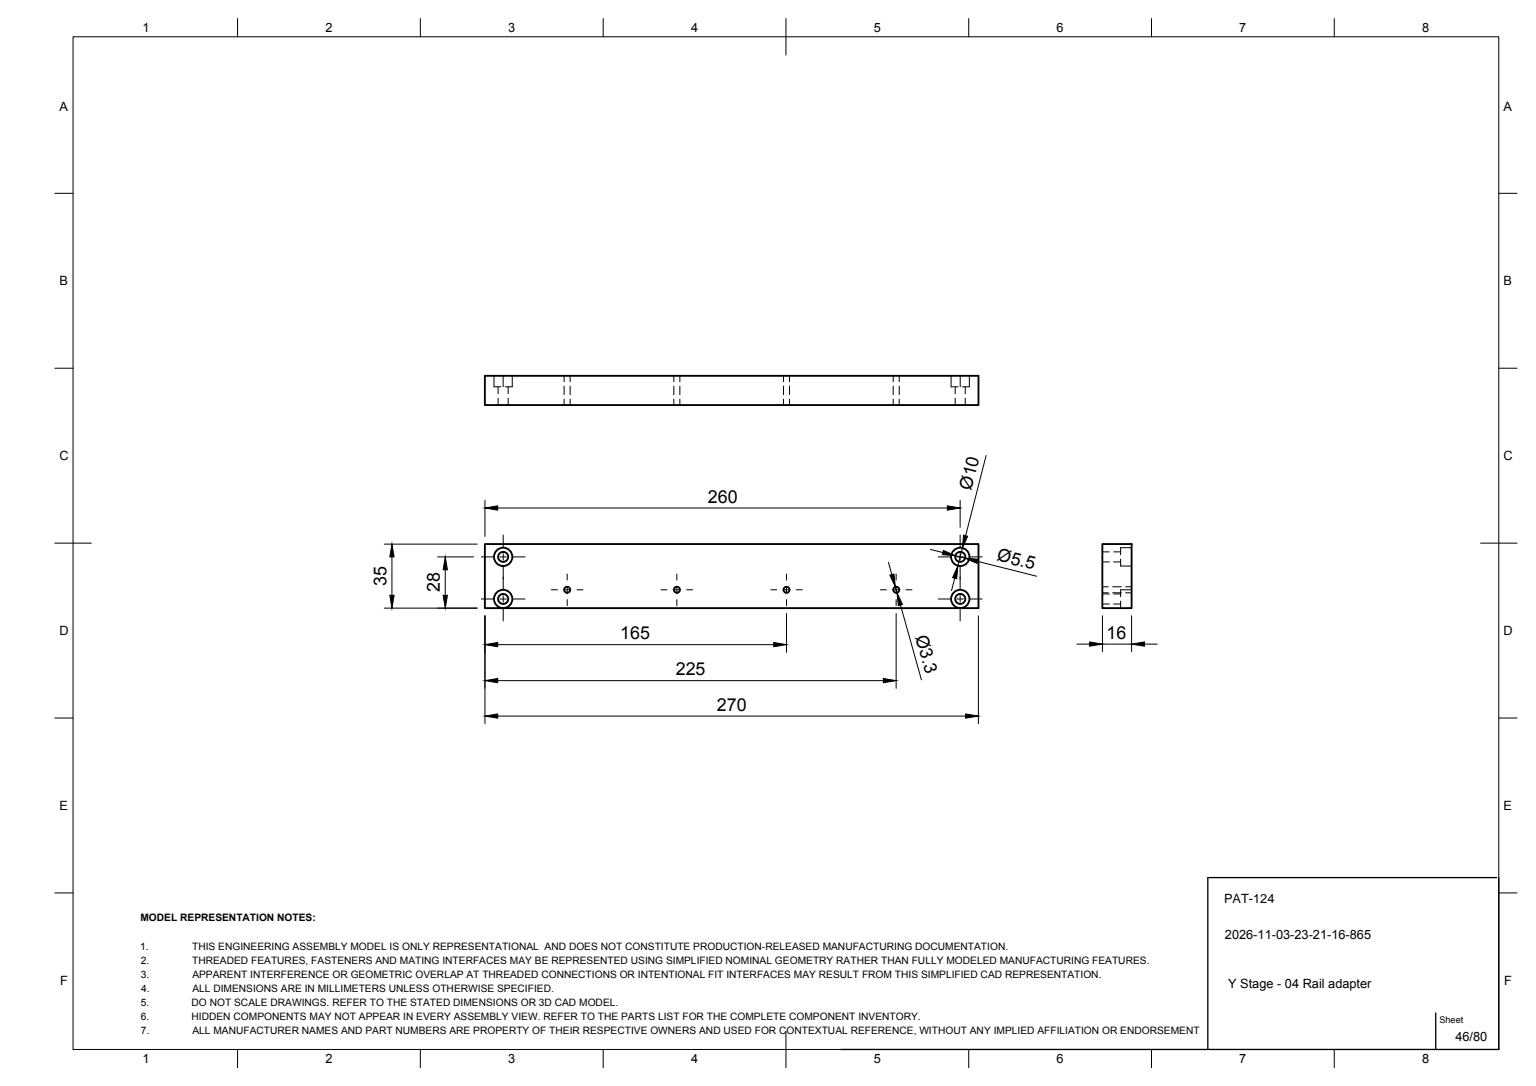
ISO-10303-21;
HEADER;
/* Generated by software containing ST-Developer
 * from STEP Tools, Inc. (www.steptools.com) 
 */

FILE_DESCRIPTION(
/* description */ ('XY cross-slide table'),
/* implementation_level */ '2;1');

FILE_NAME(
/* name */ 'Y Stage - 04 Rail adapter.step',
/* time_stamp */ '2026-10-28T03:22:46-07:00',
/* author */ (''),
/* organization */ (''),
/* preprocessor_version */ 'ST-DEVELOPER v20.2',
/* originating_system */ 'Autodesk Translation Framework v15.17.0.0',
/* authorisation */ '');

FILE_SCHEMA (('AUTOMOTIVE_DESIGN { 1 0 10303 214 3 1 1 }'));
ENDSEC;

DATA;
#10=MECHANICAL_DESIGN_GEOMETRIC_PRESENTATION_REPRESENTATION('',(#1728),#62984);
#1547=SHAPE_REPRESENTATION_RELATIONSHIP('SRR','None',#63402,#1630);
#1630=ADVANCED_BREP_SHAPE_REPRESENTATION('',(#1837),#62939);
#1728=STYLED_ITEM('',(#63905),#1837);
#1837=MANIFOLD_SOLID_BREP('Body1',#23026);
#2125=FACE_BOUND('',#5116,.T.);
#2126=FACE_BOUND('',#5119,.T.);
#2127=FACE_BOUND('',#5122,.T.);
#2128=FACE_BOUND('',#5125,.T.);
#2129=FACE_BOUND('',#5127,.T.);
#2130=FACE_BOUND('',#5128,.T.);
#2131=FACE_BOUND('',#5129,.T.);
#2132=FACE_BOUND('',#5130,.T.);
#2133=FACE_BOUND('',#5131,.T.);
#2134=FACE_BOUND('',#5132,.T.);
#2135=FACE_BOUND('',#5142,.T.);
#2136=FACE_BOUND('',#5143,.T.);
#2137=FACE_BOUND('',#5144,.T.);
#2138=FACE_BOUND('',#5145,.T.);
#2139=FACE_BOUND('',#5146,.T.);
#2140=FACE_BOUND('',#5147,.T.);
#2141=FACE_BOUND('',#5148,.T.);
#2142=FACE_BOUND('',#5149,.T.);
#2595=PLANE('',#25321);
#2596=PLANE('',#25326);
#2597=PLANE('',#25331);
#2598=PLANE('',#25336);
#2599=PLANE('',#25338);
#2600=PLANE('',#25347);
#2601=PLANE('',#25348);
#2602=PLANE('',#25349);
#2603=PLANE('',#25350);
#2604=PLANE('',#25351);
#3556=FACE_OUTER_BOUND('',#5108,.T.);
#3557=FACE_OUTER_BOUND('',#5109,.T.);
#3558=FACE_OUTER_BOUND('',#5110,.T.);
#3559=FACE_OUTER_BOUND('',#5111,.T.);
#3560=FACE_OUTER_BOUND('',#5112,.T.);
#3561=FACE_OUTER_BOUND('',#5113,.T.);
#3562=FACE_OUTER_BOUND('',#5114,.T.);
#3563=FACE_OUTER_BOUND('',#5115,.T.);
#3564=FACE_OUTER_BOUND('',#5117,.T.);
#3565=FACE_OUTER_BOUND('',#5118,.T.);
#3566=FACE_OUTER_BOUND('',#5120,.T.);
#3567=FACE_OUTER_BOUND('',#5121,.T.);
#3568=FACE_OUTER_BOUND('',#5123,.T.);
#3569=FACE_OUTER_BOUND('',#5124,.T.);
#3570=FACE_OUTER_BOUND('',#5126,.T.);
#3571=FACE_OUTER_BOUND('',#5133,.T.);
#3572=FACE_OUTER_BOUND('',#5134,.T.);
#3573=FACE_OUTER_BOUND('',#5135,.T.);
#3574=FACE_OUTER_BOUND('',#5136,.T.);
#3575=FACE_OUTER_BOUND('',#5137,.T.);
#3576=FACE_OUTER_BOUND('',#5138,.T.);
#3577=FACE_OUTER_BOUND('',#5139,.T.);
#3578=FACE_OUTER_BOUND('',#5140,.T.);
#3579=FACE_OUTER_BOUND('',#5141,.T.);
#5108=EDGE_LOOP('',(#18110,#18111,#18112,#18113));
#5109=EDGE_LOOP('',(#18114,#18115,#18116,#18117));
#5110=EDGE_LOOP('',(#18118,#18119,#18120,#18121));
#5111=EDGE_LOOP('',(#18122,#18123,#18124,#18125));
#5112=EDGE_LOOP('',(#18126,#18127,#18128,#18129));
#5113=EDGE_LOOP('',(#18130,#18131,#18132,#18133));
#5114=EDGE_LOOP('',(#18134,#18135,#18136,#18137));
#5115=EDGE_LOOP('',(#18138));
#5116=EDGE_LOOP('',(#18139));
#5117=EDGE_LOOP('',(#18140,#18141,#18142,#18143));
#5118=EDGE_LOOP('',(#18144,#18145));
#5119=EDGE_LOOP('',(#18146));
#5120=EDGE_LOOP('',(#18147,#18148,#18149,#18150));
#5121=EDGE_LOOP('',(#18151));
#5122=EDGE_LOOP('',(#18152));
#5123=EDGE_LOOP('',(#18153,#18154,#18155,#18156));
#5124=EDGE_LOOP('',(#18157,#18158));
#5125=EDGE_LOOP('',(#18159));
#5126=EDGE_LOOP('',(#18160,#18161,#18162,#18163,#18164,#18165,#18166,#18167,
#18168,#18169));
#5127=EDGE_LOOP('',(#18170));
#5128=EDGE_LOOP('',(#18171));
#5129=EDGE_LOOP('',(#18172));
#5130=EDGE_LOOP('',(#18173));
#5131=EDGE_LOOP('',(#18174));
#5132=EDGE_LOOP('',(#18175));
#5133=EDGE_LOOP('',(#18176,#18177,#18178,#18179));
#5134=EDGE_LOOP('',(#18180,#18181,#18182,#18183));
#5135=EDGE_LOOP('',(#18184,#18185,#18186,#18187));
#5136=EDGE_LOOP('',(#18188,#18189,#18190,#18191));
#5137=EDGE_LOOP('',(#18192,#18193,#18194,#18195,#18196,#18197,#18198,#18199,
#18200,#18201));
#5138=EDGE_LOOP('',(#18202,#18203,#18204,#18205));
#5139=EDGE_LOOP('',(#18206,#18207,#18208,#18209));
#5140=EDGE_LOOP('',(#18210,#18211,#18212,#18213));
#5141=EDGE_LOOP('',(#18214,#18215,#18216,#18217));
#5142=EDGE_LOOP('',(#18218));
#5143=EDGE_LOOP('',(#18219));
#5144=EDGE_LOOP('',(#18220));
#5145=EDGE_LOOP('',(#18221));
#5146=EDGE_LOOP('',(#18222));
#5147=EDGE_LOOP('',(#18223));
#5148=EDGE_LOOP('',(#18224));
#5149=EDGE_LOOP('',(#18225));
#6682=LINE('',#47980,#8169);
#6683=LINE('',#47984,#8170);
#6684=LINE('',#47989,#8171);
#6685=LINE('',#47993,#8172);
#6686=LINE('',#47999,#8173);
#6687=LINE('',#48005,#8174);
#6688=LINE('',#48011,#8175);
#6689=LINE('',#48017,#8176);
#6690=LINE('',#48023,#8177);
#6691=LINE('',#48030,#8178);
#6692=LINE('',#48039,#8179);
#6693=LINE('',#48046,#8180);
#6694=LINE('',#48054,#8181);
#6695=LINE('',#48056,#8182);
#6696=LINE('',#48058,#8183);
#6697=LINE('',#48059,#8184);
#6698=LINE('',#48060,#8185);
#6699=LINE('',#48061,#8186);
#6700=LINE('',#48065,#8187);
#6701=LINE('',#48069,#8188);
#6702=LINE('',#48073,#8189);
#6703=LINE('',#48077,#8190);
#6704=LINE('',#48081,#8191);
#6705=LINE('',#48082,#8192);
#6706=LINE('',#48083,#8193);
#6707=LINE('',#48086,#8194);
#6708=LINE('',#48087,#8195);
#6709=LINE('',#48090,#8196);
#6710=LINE('',#48091,#8197);
#6711=LINE('',#48093,#8198);
#8169=VECTOR('',#29839,0.5);
#8170=VECTOR('',#29842,1.);
#8171=VECTOR('',#29847,0.5);
#8172=VECTOR('',#29850,1.);
#8173=VECTOR('',#29857,0.164999999999999);
#8174=VECTOR('',#29864,0.164999999999999);
#8175=VECTOR('',#29871,0.165);
#8176=VECTOR('',#29878,0.164999999999999);
#8177=VECTOR('',#29885,0.5);
#8178=VECTOR('',#29896,1.);
#8179=VECTOR('',#29907,0.5);
#8180=VECTOR('',#29918,1.);
#8181=VECTOR('',#29927,1.);
#8182=VECTOR('',#29928,1.);
#8183=VECTOR('',#29929,1.);
#8184=VECTOR('',#29930,1.);
#8185=VECTOR('',#29931,1.);
#8186=VECTOR('',#29932,1.);
#8187=VECTOR('',#29937,0.274999999999999);
#8188=VECTOR('',#29942,0.275);
#8189=VECTOR('',#29947,0.275);
#8190=VECTOR('',#29952,0.274999999999999);
#8191=VECTOR('',#29955,1.);
#8192=VECTOR('',#29956,1.);
#8193=VECTOR('',#29957,1.);
#8194=VECTOR('',#29960,1.);
#8195=VECTOR('',#29961,1.);
#8196=VECTOR('',#29964,1.);
#8197=VECTOR('',#29965,1.);
#8198=VECTOR('',#29968,1.);
#9363=CIRCLE('',#25301,0.5);
#9364=CIRCLE('',#25302,0.5);
#9365=CIRCLE('',#25304,0.5);
#9366=CIRCLE('',#25305,0.5);
#9367=CIRCLE('',#25307,0.164999999999999);
#9368=CIRCLE('',#25308,0.164999999999999);
#9369=CIRCLE('',#25310,0.164999999999999);
#9370=CIRCLE('',#25311,0.164999999999999);
#9371=CIRCLE('',#25313,0.165);
#9372=CIRCLE('',#25314,0.165);
#9373=CIRCLE('',#25316,0.164999999999999);
#9374=CIRCLE('',#25317,0.164999999999999);
#9375=CIRCLE('',#25319,0.5);
#9376=CIRCLE('',#25320,0.5);
#9377=CIRCLE('',#25322,0.274999999999999);
#9378=CIRCLE('',#25324,0.5);
#9379=CIRCLE('',#25325,0.5);
#9380=CIRCLE('',#25327,0.275);
#9381=CIRCLE('',#25329,0.5);
#9382=CIRCLE('',#25330,0.5);
#9383=CIRCLE('',#25332,0.275);
#9384=CIRCLE('',#25334,0.5);
#9385=CIRCLE('',#25335,0.5);
#9386=CIRCLE('',#25337,0.274999999999999);
#9387=CIRCLE('',#25340,0.274999999999999);
#9388=CIRCLE('',#25342,0.275);
#9389=CIRCLE('',#25344,0.275);
#9390=CIRCLE('',#25346,0.274999999999999);
#10851=VERTEX_POINT('',#47978);
#10852=VERTEX_POINT('',#47979);
#10853=VERTEX_POINT('',#47981);
#10854=VERTEX_POINT('',#47983);
#10855=VERTEX_POINT('',#47987);
#10856=VERTEX_POINT('',#47988);
#10857=VERTEX_POINT('',#47990);
#10858=VERTEX_POINT('',#47992);
#10859=VERTEX_POINT('',#47996);
#10860=VERTEX_POINT('',#47998);
#10861=VERTEX_POINT('',#48002);
#10862=VERTEX_POINT('',#48004);
#10863=VERTEX_POINT('',#48008);
#10864=VERTEX_POINT('',#48010);
#10865=VERTEX_POINT('',#48014);
#10866=VERTEX_POINT('',#48016);
#10867=VERTEX_POINT('',#48020);
#10868=VERTEX_POINT('',#48022);
#10869=VERTEX_POINT('',#48026);
#10870=VERTEX_POINT('',#48033);
#10871=VERTEX_POINT('',#48036);
#10872=VERTEX_POINT('',#48038);
#10873=VERTEX_POINT('',#48042);
#10874=VERTEX_POINT('',#48049);
#10875=VERTEX_POINT('',#48052);
#10876=VERTEX_POINT('',#48053);
#10877=VERTEX_POINT('',#48055);
#10878=VERTEX_POINT('',#48057);
#10879=VERTEX_POINT('',#48063);
#10880=VERTEX_POINT('',#48067);
#10881=VERTEX_POINT('',#48071);
#10882=VERTEX_POINT('',#48075);
#10883=VERTEX_POINT('',#48079);
#10884=VERTEX_POINT('',#48080);
#10885=VERTEX_POINT('',#48085);
#10886=VERTEX_POINT('',#48089);
#13439=EDGE_CURVE('',#10851,#10852,#6682,.T.);
#13440=EDGE_CURVE('',#10853,#10851,#9363,.T.);
#13441=EDGE_CURVE('',#10853,#10854,#6683,.T.);
#13442=EDGE_CURVE('',#10852,#10854,#9364,.T.);
#13443=EDGE_CURVE('',#10855,#10856,#6684,.T.);
#13444=EDGE_CURVE('',#10857,#10855,#9365,.T.);
#13445=EDGE_CURVE('',#10857,#10858,#6685,.T.);
#13446=EDGE_CURVE('',#10856,#10858,#9366,.T.);
#13447=EDGE_CURVE('',#10859,#10859,#9367,.T.);
#13448=EDGE_CURVE('',#10859,#10860,#6686,.T.);
#13449=EDGE_CURVE('',#10860,#10860,#9368,.T.);
#13450=EDGE_CURVE('',#10861,#10861,#9369,.T.);
#13451=EDGE_CURVE('',#10861,#10862,#6687,.T.);
#13452=EDGE_CURVE('',#10862,#10862,#9370,.T.);
#13453=EDGE_CURVE('',#10863,#10863,#9371,.T.);
#13454=EDGE_CURVE('',#10863,#10864,#6688,.T.);
#13455=EDGE_CURVE('',#10864,#10864,#9372,.T.);
#13456=EDGE_CURVE('',#10865,#10865,#9373,.T.);
#13457=EDGE_CURVE('',#10865,#10866,#6689,.T.);
#13458=EDGE_CURVE('',#10866,#10866,#9374,.T.);
#13459=EDGE_CURVE('',#10867,#10867,#9375,.T.);
#13460=EDGE_CURVE('',#10867,#10868,#6690,.T.);
#13461=EDGE_CURVE('',#10868,#10868,#9376,.T.);
#13462=EDGE_CURVE('',#10869,#10869,#9377,.T.);
#13463=EDGE_CURVE('',#10858,#10856,#9378,.T.);
#13464=EDGE_CURVE('',#10857,#10858,#6691,.T.);
#13465=EDGE_CURVE('',#10855,#10857,#9379,.T.);
#13466=EDGE_CURVE('',#10870,#10870,#9380,.T.);
#13467=EDGE_CURVE('',#10871,#10871,#9381,.T.);
#13468=EDGE_CURVE('',#10871,#10872,#6692,.T.);
#13469=EDGE_CURVE('',#10872,#10872,#9382,.T.);
#13470=EDGE_CURVE('',#10873,#10873,#9383,.T.);
#13471=EDGE_CURVE('',#10854,#10852,#9384,.T.);
#13472=EDGE_CURVE('',#10853,#10854,#6693,.T.);
#13473=EDGE_CURVE('',#10851,#10853,#9385,.T.);
#13474=EDGE_CURVE('',#10874,#10874,#9386,.T.);
#13475=EDGE_CURVE('',#10875,#10876,#6694,.T.);
#13476=EDGE_CURVE('',#10876,#10877,#6695,.T.);
#13477=EDGE_CURVE('',#10877,#10878,#6696,.T.);
#13478=EDGE_CURVE('',#10878,#10854,#6697,.T.);
#13479=EDGE_CURVE('',#10854,#10858,#6698,.T.);
#13480=EDGE_CURVE('',#10858,#10875,#6699,.T.);
#13481=EDGE_CURVE('',#10879,#10879,#9387,.T.);
#13482=EDGE_CURVE('',#10879,#10869,#6700,.T.);
#13483=EDGE_CURVE('',#10880,#10880,#9388,.T.);
#13484=EDGE_CURVE('',#10880,#10870,#6701,.T.);
#13485=EDGE_CURVE('',#10881,#10881,#9389,.T.);
#13486=EDGE_CURVE('',#10881,#10873,#6702,.T.);
#13487=EDGE_CURVE('',#10882,#10882,#9390,.T.);
#13488=EDGE_CURVE('',#10882,#10874,#6703,.T.);
#13489=EDGE_CURVE('',#10883,#10884,#6704,.T.);
#13490=EDGE_CURVE('',#10884,#10875,#6705,.T.);
#13491=EDGE_CURVE('',#10883,#10878,#6706,.T.);
#13492=EDGE_CURVE('',#10885,#10883,#6707,.T.);
#13493=EDGE_CURVE('',#10885,#10877,#6708,.T.);
#13494=EDGE_CURVE('',#10886,#10885,#6709,.T.);
#13495=EDGE_CURVE('',#10886,#10876,#6710,.T.);
#13496=EDGE_CURVE('',#10884,#10886,#6711,.T.);
#18110=ORIENTED_EDGE('',*,*,#13439,.F.);
#18111=ORIENTED_EDGE('',*,*,#13440,.F.);
#18112=ORIENTED_EDGE('',*,*,#13441,.T.);
#18113=ORIENTED_EDGE('',*,*,#13442,.F.);
#18114=ORIENTED_EDGE('',*,*,#13443,.F.);
#18115=ORIENTED_EDGE('',*,*,#13444,.F.);
#18116=ORIENTED_EDGE('',*,*,#13445,.T.);
#18117=ORIENTED_EDGE('',*,*,#13446,.F.);
#18118=ORIENTED_EDGE('',*,*,#13447,.F.);
#18119=ORIENTED_EDGE('',*,*,#13448,.T.);
#18120=ORIENTED_EDGE('',*,*,#13449,.F.);
#18121=ORIENTED_EDGE('',*,*,#13448,.F.);
#18122=ORIENTED_EDGE('',*,*,#13450,.F.);
#18123=ORIENTED_EDGE('',*,*,#13451,.T.);
#18124=ORIENTED_EDGE('',*,*,#13452,.F.);
#18125=ORIENTED_EDGE('',*,*,#13451,.F.);
#18126=ORIENTED_EDGE('',*,*,#13453,.F.);
#18127=ORIENTED_EDGE('',*,*,#13454,.T.);
#18128=ORIENTED_EDGE('',*,*,#13455,.F.);
#18129=ORIENTED_EDGE('',*,*,#13454,.F.);
#18130=ORIENTED_EDGE('',*,*,#13456,.F.);
#18131=ORIENTED_EDGE('',*,*,#13457,.T.);
#18132=ORIENTED_EDGE('',*,*,#13458,.F.);
#18133=ORIENTED_EDGE('',*,*,#13457,.F.);
#18134=ORIENTED_EDGE('',*,*,#13459,.F.);
#18135=ORIENTED_EDGE('',*,*,#13460,.T.);
#18136=ORIENTED_EDGE('',*,*,#13461,.F.);
#18137=ORIENTED_EDGE('',*,*,#13460,.F.);
#18138=ORIENTED_EDGE('',*,*,#13459,.T.);
#18139=ORIENTED_EDGE('',*,*,#13462,.F.);
#18140=ORIENTED_EDGE('',*,*,#13443,.T.);
#18141=ORIENTED_EDGE('',*,*,#13463,.F.);
#18142=ORIENTED_EDGE('',*,*,#13464,.F.);
#18143=ORIENTED_EDGE('',*,*,#13465,.F.);
#18144=ORIENTED_EDGE('',*,*,#13444,.T.);
#18145=ORIENTED_EDGE('',*,*,#13465,.T.);
#18146=ORIENTED_EDGE('',*,*,#13466,.F.);
#18147=ORIENTED_EDGE('',*,*,#13467,.F.);
#18148=ORIENTED_EDGE('',*,*,#13468,.T.);
#18149=ORIENTED_EDGE('',*,*,#13469,.F.);
#18150=ORIENTED_EDGE('',*,*,#13468,.F.);
#18151=ORIENTED_EDGE('',*,*,#13467,.T.);
#18152=ORIENTED_EDGE('',*,*,#13470,.F.);
#18153=ORIENTED_EDGE('',*,*,#13439,.T.);
#18154=ORIENTED_EDGE('',*,*,#13471,.F.);
#18155=ORIENTED_EDGE('',*,*,#13472,.F.);
#18156=ORIENTED_EDGE('',*,*,#13473,.F.);
#18157=ORIENTED_EDGE('',*,*,#13440,.T.);
#18158=ORIENTED_EDGE('',*,*,#13473,.T.);
#18159=ORIENTED_EDGE('',*,*,#13474,.F.);
#18160=ORIENTED_EDGE('',*,*,#13475,.T.);
#18161=ORIENTED_EDGE('',*,*,#13476,.T.);
#18162=ORIENTED_EDGE('',*,*,#13477,.T.);
#18163=ORIENTED_EDGE('',*,*,#13478,.T.);
#18164=ORIENTED_EDGE('',*,*,#13471,.T.);
#18165=ORIENTED_EDGE('',*,*,#13442,.T.);
#18166=ORIENTED_EDGE('',*,*,#13479,.T.);
#18167=ORIENTED_EDGE('',*,*,#13463,.T.);
#18168=ORIENTED_EDGE('',*,*,#13446,.T.);
#18169=ORIENTED_EDGE('',*,*,#13480,.T.);
#18170=ORIENTED_EDGE('',*,*,#13461,.T.);
#18171=ORIENTED_EDGE('',*,*,#13469,.T.);
#18172=ORIENTED_EDGE('',*,*,#13458,.T.);
#18173=ORIENTED_EDGE('',*,*,#13455,.T.);
#18174=ORIENTED_EDGE('',*,*,#13452,.T.);
#18175=ORIENTED_EDGE('',*,*,#13449,.T.);
#18176=ORIENTED_EDGE('',*,*,#13481,.F.);
#18177=ORIENTED_EDGE('',*,*,#13482,.T.);
#18178=ORIENTED_EDGE('',*,*,#13462,.T.);
#18179=ORIENTED_EDGE('',*,*,#13482,.F.);
#18180=ORIENTED_EDGE('',*,*,#13483,.F.);
#18181=ORIENTED_EDGE('',*,*,#13484,.T.);
#18182=ORIENTED_EDGE('',*,*,#13466,.T.);
#18183=ORIENTED_EDGE('',*,*,#13484,.F.);
#18184=ORIENTED_EDGE('',*,*,#13485,.F.);
#18185=ORIENTED_EDGE('',*,*,#13486,.T.);
#18186=ORIENTED_EDGE('',*,*,#13470,.T.);
#18187=ORIENTED_EDGE('',*,*,#13486,.F.);
#18188=ORIENTED_EDGE('',*,*,#13487,.F.);
#18189=ORIENTED_EDGE('',*,*,#13488,.T.);
#18190=ORIENTED_EDGE('',*,*,#13474,.T.);
#18191=ORIENTED_EDGE('',*,*,#13488,.F.);
#18192=ORIENTED_EDGE('',*,*,#13489,.T.);
#18193=ORIENTED_EDGE('',*,*,#13490,.T.);
#18194=ORIENTED_EDGE('',*,*,#13480,.F.);
#18195=ORIENTED_EDGE('',*,*,#13445,.F.);
#18196=ORIENTED_EDGE('',*,*,#13464,.T.);
#18197=ORIENTED_EDGE('',*,*,#13479,.F.);
#18198=ORIENTED_EDGE('',*,*,#13441,.F.);
#18199=ORIENTED_EDGE('',*,*,#13472,.T.);
#18200=ORIENTED_EDGE('',*,*,#13478,.F.);
#18201=ORIENTED_EDGE('',*,*,#13491,.F.);
#18202=ORIENTED_EDGE('',*,*,#13492,.T.);
#18203=ORIENTED_EDGE('',*,*,#13491,.T.);
#18204=ORIENTED_EDGE('',*,*,#13477,.F.);
#18205=ORIENTED_EDGE('',*,*,#13493,.F.);
#18206=ORIENTED_EDGE('',*,*,#13494,.T.);
#18207=ORIENTED_EDGE('',*,*,#13493,.T.);
#18208=ORIENTED_EDGE('',*,*,#13476,.F.);
#18209=ORIENTED_EDGE('',*,*,#13495,.F.);
#18210=ORIENTED_EDGE('',*,*,#13496,.T.);
#18211=ORIENTED_EDGE('',*,*,#13495,.T.);
#18212=ORIENTED_EDGE('',*,*,#13475,.F.);
#18213=ORIENTED_EDGE('',*,*,#13490,.F.);
#18214=ORIENTED_EDGE('',*,*,#13496,.F.);
#18215=ORIENTED_EDGE('',*,*,#13489,.F.);
#18216=ORIENTED_EDGE('',*,*,#13492,.F.);
#18217=ORIENTED_EDGE('',*,*,#13494,.F.);
#18218=ORIENTED_EDGE('',*,*,#13487,.T.);
#18219=ORIENTED_EDGE('',*,*,#13485,.T.);
#18220=ORIENTED_EDGE('',*,*,#13483,.T.);
#18221=ORIENTED_EDGE('',*,*,#13481,.T.);
#18222=ORIENTED_EDGE('',*,*,#13456,.T.);
#18223=ORIENTED_EDGE('',*,*,#13453,.T.);
#18224=ORIENTED_EDGE('',*,*,#13450,.T.);
#18225=ORIENTED_EDGE('',*,*,#13447,.T.);
#21364=CYLINDRICAL_SURFACE('',#25300,0.5);
#21365=CYLINDRICAL_SURFACE('',#25303,0.5);
#21366=CYLINDRICAL_SURFACE('',#25306,0.164999999999999);
#21367=CYLINDRICAL_SURFACE('',#25309,0.164999999999999);
#21368=CYLINDRICAL_SURFACE('',#25312,0.165);
#21369=CYLINDRICAL_SURFACE('',#25315,0.164999999999999);
#21370=CYLINDRICAL_SURFACE('',#25318,0.5);
#21371=CYLINDRICAL_SURFACE('',#25323,0.5);
#21372=CYLINDRICAL_SURFACE('',#25328,0.5);
#21373=CYLINDRICAL_SURFACE('',#25333,0.5);
#21374=CYLINDRICAL_SURFACE('',#25339,0.274999999999999);
#21375=CYLINDRICAL_SURFACE('',#25341,0.275);
#21376=CYLINDRICAL_SURFACE('',#25343,0.275);
#21377=CYLINDRICAL_SURFACE('',#25345,0.274999999999999);
#22337=ADVANCED_FACE('',(#3556),#21364,.F.);
#22338=ADVANCED_FACE('',(#3557),#21365,.F.);
#22339=ADVANCED_FACE('',(#3558),#21366,.F.);
#22340=ADVANCED_FACE('',(#3559),#21367,.F.);
#22341=ADVANCED_FACE('',(#3560),#21368,.F.);
#22342=ADVANCED_FACE('',(#3561),#21369,.F.);
#22343=ADVANCED_FACE('',(#3562),#21370,.F.);
#22344=ADVANCED_FACE('',(#3563,#2125),#2595,.T.);
#22345=ADVANCED_FACE('',(#3564),#21371,.F.);
#22346=ADVANCED_FACE('',(#3565,#2126),#2596,.T.);
#22347=ADVANCED_FACE('',(#3566),#21372,.F.);
#22348=ADVANCED_FACE('',(#3567,#2127),#2597,.T.);
#22349=ADVANCED_FACE('',(#3568),#21373,.F.);
#22350=ADVANCED_FACE('',(#3569,#2128),#2598,.T.);
#22351=ADVANCED_FACE('',(#3570,#2129,#2130,#2131,#2132,#2133,#2134),#2599,
 .T.);
#22352=ADVANCED_FACE('',(#3571),#21374,.F.);
#22353=ADVANCED_FACE('',(#3572),#21375,.F.);
#22354=ADVANCED_FACE('',(#3573),#21376,.F.);
#22355=ADVANCED_FACE('',(#3574),#21377,.F.);
#22356=ADVANCED_FACE('',(#3575),#2600,.T.);
#22357=ADVANCED_FACE('',(#3576),#2601,.T.);
#22358=ADVANCED_FACE('',(#3577),#2602,.T.);
#22359=ADVANCED_FACE('',(#3578),#2603,.T.);
#22360=ADVANCED_FACE('',(#3579,#2135,#2136,#2137,#2138,#2139,#2140,#2141,
#2142),#2604,.F.);
#23026=CLOSED_SHELL('',(#22337,#22338,#22339,#22340,#22341,#22342,#22343,
#22344,#22345,#22346,#22347,#22348,#22349,#22350,#22351,#22352,#22353,#22354,
#22355,#22356,#22357,#22358,#22359,#22360));
#25299=AXIS2_PLACEMENT_3D('',#47976,#29835,#29836);
#25300=AXIS2_PLACEMENT_3D('',#47977,#29837,#29838);
#25301=AXIS2_PLACEMENT_3D('',#47982,#29840,#29841);
#25302=AXIS2_PLACEMENT_3D('',#47985,#29843,#29844);
#25303=AXIS2_PLACEMENT_3D('',#47986,#29845,#29846);
#25304=AXIS2_PLACEMENT_3D('',#47991,#29848,#29849);
#25305=AXIS2_PLACEMENT_3D('',#47994,#29851,#29852);
#25306=AXIS2_PLACEMENT_3D('',#47995,#29853,#29854);
#25307=AXIS2_PLACEMENT_3D('',#47997,#29855,#29856);
#25308=AXIS2_PLACEMENT_3D('',#48000,#29858,#29859);
#25309=AXIS2_PLACEMENT_3D('',#48001,#29860,#29861);
#25310=AXIS2_PLACEMENT_3D('',#48003,#29862,#29863);
#25311=AXIS2_PLACEMENT_3D('',#48006,#29865,#29866);
#25312=AXIS2_PLACEMENT_3D('',#48007,#29867,#29868);
#25313=AXIS2_PLACEMENT_3D('',#48009,#29869,#29870);
#25314=AXIS2_PLACEMENT_3D('',#48012,#29872,#29873);
#25315=AXIS2_PLACEMENT_3D('',#48013,#29874,#29875);
#25316=AXIS2_PLACEMENT_3D('',#48015,#29876,#29877);
#25317=AXIS2_PLACEMENT_3D('',#48018,#29879,#29880);
#25318=AXIS2_PLACEMENT_3D('',#48019,#29881,#29882);
#25319=AXIS2_PLACEMENT_3D('',#48021,#29883,#29884);
#25320=AXIS2_PLACEMENT_3D('',#48024,#29886,#29887);
#25321=AXIS2_PLACEMENT_3D('',#48025,#29888,#29889);
#25322=AXIS2_PLACEMENT_3D('',#48027,#29890,#29891);
#25323=AXIS2_PLACEMENT_3D('',#48028,#29892,#29893);
#25324=AXIS2_PLACEMENT_3D('',#48029,#29894,#29895);
#25325=AXIS2_PLACEMENT_3D('',#48031,#29897,#29898);
#25326=AXIS2_PLACEMENT_3D('',#48032,#29899,#29900);
#25327=AXIS2_PLACEMENT_3D('',#48034,#29901,#29902);
#25328=AXIS2_PLACEMENT_3D('',#48035,#29903,#29904);
#25329=AXIS2_PLACEMENT_3D('',#48037,#29905,#29906);
#25330=AXIS2_PLACEMENT_3D('',#48040,#29908,#29909);
#25331=AXIS2_PLACEMENT_3D('',#48041,#29910,#29911);
#25332=AXIS2_PLACEMENT_3D('',#48043,#29912,#29913);
#25333=AXIS2_PLACEMENT_3D('',#48044,#29914,#29915);
#25334=AXIS2_PLACEMENT_3D('',#48045,#29916,#29917);
#25335=AXIS2_PLACEMENT_3D('',#48047,#29919,#29920);
#25336=AXIS2_PLACEMENT_3D('',#48048,#29921,#29922);
#25337=AXIS2_PLACEMENT_3D('',#48050,#29923,#29924);
#25338=AXIS2_PLACEMENT_3D('',#48051,#29925,#29926);
#25339=AXIS2_PLACEMENT_3D('',#48062,#29933,#29934);
#25340=AXIS2_PLACEMENT_3D('',#48064,#29935,#29936);
#25341=AXIS2_PLACEMENT_3D('',#48066,#29938,#29939);
#25342=AXIS2_PLACEMENT_3D('',#48068,#29940,#29941);
#25343=AXIS2_PLACEMENT_3D('',#48070,#29943,#29944);
#25344=AXIS2_PLACEMENT_3D('',#48072,#29945,#29946);
#25345=AXIS2_PLACEMENT_3D('',#48074,#29948,#29949);
#25346=AXIS2_PLACEMENT_3D('',#48076,#29950,#29951);
#25347=AXIS2_PLACEMENT_3D('',#48078,#29953,#29954);
#25348=AXIS2_PLACEMENT_3D('',#48084,#29958,#29959);
#25349=AXIS2_PLACEMENT_3D('',#48088,#29962,#29963);
#25350=AXIS2_PLACEMENT_3D('',#48092,#29966,#29967);
#25351=AXIS2_PLACEMENT_3D('',#48094,#29969,#29970);
#29835=DIRECTION('axis',(0.,0.,1.));
#29836=DIRECTION('refdir',(1.,0.,0.));
#29837=DIRECTION('center_axis',(0.,0.,1.));
#29838=DIRECTION('ref_axis',(1.,0.,0.));
#29839=DIRECTION('',(0.,0.,1.));
#29840=DIRECTION('center_axis',(0.,0.,1.));
#29841=DIRECTION('ref_axis',(1.,0.,0.));
#29842=DIRECTION('',(0.,0.,1.));
#29843=DIRECTION('center_axis',(0.,0.,-1.));
#29844=DIRECTION('ref_axis',(1.,0.,0.));
#29845=DIRECTION('center_axis',(0.,0.,1.));
#29846=DIRECTION('ref_axis',(1.,0.,0.));
#29847=DIRECTION('',(0.,0.,1.));
#29848=DIRECTION('center_axis',(0.,0.,1.));
#29849=DIRECTION('ref_axis',(1.,0.,0.));
#29850=DIRECTION('',(0.,0.,1.));
#29851=DIRECTION('center_axis',(0.,0.,-1.));
#29852=DIRECTION('ref_axis',(1.,0.,0.));
#29853=DIRECTION('center_axis',(0.,0.,1.));
#29854=DIRECTION('ref_axis',(1.,0.,0.));
#29855=DIRECTION('center_axis',(0.,0.,1.));
#29856=DIRECTION('ref_axis',(1.,0.,0.));
#29857=DIRECTION('',(0.,0.,1.));
#29858=DIRECTION('center_axis',(0.,0.,-1.));
#29859=DIRECTION('ref_axis',(1.,0.,0.));
#29860=DIRECTION('center_axis',(0.,0.,1.));
#29861=DIRECTION('ref_axis',(1.,0.,0.));
#29862=DIRECTION('center_axis',(0.,0.,1.));
#29863=DIRECTION('ref_axis',(1.,0.,0.));
#29864=DIRECTION('',(0.,0.,1.));
#29865=DIRECTION('center_axis',(0.,0.,-1.));
#29866=DIRECTION('ref_axis',(1.,0.,0.));
#29867=DIRECTION('center_axis',(0.,0.,1.));
#29868=DIRECTION('ref_axis',(1.,0.,0.));
#29869=DIRECTION('center_axis',(0.,0.,1.));
#29870=DIRECTION('ref_axis',(1.,0.,0.));
#29871=DIRECTION('',(0.,0.,1.));
#29872=DIRECTION('center_axis',(0.,0.,-1.));
#29873=DIRECTION('ref_axis',(1.,0.,0.));
#29874=DIRECTION('center_axis',(0.,0.,1.));
#29875=DIRECTION('ref_axis',(1.,0.,0.));
#29876=DIRECTION('center_axis',(0.,0.,1.));
#29877=DIRECTION('ref_axis',(1.,0.,0.));
#29878=DIRECTION('',(0.,0.,1.));
#29879=DIRECTION('center_axis',(0.,0.,-1.));
#29880=DIRECTION('ref_axis',(1.,0.,0.));
#29881=DIRECTION('center_axis',(0.,0.,1.));
#29882=DIRECTION('ref_axis',(1.,0.,0.));
#29883=DIRECTION('center_axis',(0.,0.,1.));
#29884=DIRECTION('ref_axis',(1.,0.,0.));
#29885=DIRECTION('',(0.,0.,1.));
#29886=DIRECTION('center_axis',(0.,0.,-1.));
#29887=DIRECTION('ref_axis',(1.,0.,0.));
#29888=DIRECTION('center_axis',(0.,0.,1.));
#29889=DIRECTION('ref_axis',(1.,0.,0.));
#29890=DIRECTION('center_axis',(0.,0.,1.));
#29891=DIRECTION('ref_axis',(1.,0.,0.));
#29892=DIRECTION('center_axis',(0.,0.,1.));
#29893=DIRECTION('ref_axis',(1.,0.,0.));
#29894=DIRECTION('center_axis',(0.,0.,-1.));
#29895=DIRECTION('ref_axis',(1.,0.,0.));
#29896=DIRECTION('',(0.,0.,1.));
#29897=DIRECTION('center_axis',(0.,0.,1.));
#29898=DIRECTION('ref_axis',(1.,0.,0.));
#29899=DIRECTION('center_axis',(0.,0.,1.));
#29900=DIRECTION('ref_axis',(1.,0.,0.));
#29901=DIRECTION('center_axis',(0.,0.,1.));
#29902=DIRECTION('ref_axis',(1.,0.,0.));
#29903=DIRECTION('center_axis',(0.,0.,1.));
#29904=DIRECTION('ref_axis',(1.,0.,0.));
#29905=DIRECTION('center_axis',(0.,0.,1.));
#29906=DIRECTION('ref_axis',(1.,0.,0.));
#29907=DIRECTION('',(0.,0.,1.));
#29908=DIRECTION('center_axis',(0.,0.,-1.));
#29909=DIRECTION('ref_axis',(1.,0.,0.));
#29910=DIRECTION('center_axis',(0.,0.,1.));
#29911=DIRECTION('ref_axis',(1.,0.,0.));
#29912=DIRECTION('center_axis',(0.,0.,1.));
#29913=DIRECTION('ref_axis',(1.,0.,0.));
#29914=DIRECTION('center_axis',(0.,0.,1.));
#29915=DIRECTION('ref_axis',(1.,0.,0.));
#29916=DIRECTION('center_axis',(0.,0.,-1.));
#29917=DIRECTION('ref_axis',(1.,0.,0.));
#29918=DIRECTION('',(0.,0.,1.));
#29919=DIRECTION('center_axis',(0.,0.,1.));
#29920=DIRECTION('ref_axis',(1.,0.,0.));
#29921=DIRECTION('center_axis',(0.,0.,1.));
#29922=DIRECTION('ref_axis',(1.,0.,0.));
#29923=DIRECTION('center_axis',(0.,0.,1.));
#29924=DIRECTION('ref_axis',(1.,0.,0.));
#29925=DIRECTION('center_axis',(0.,0.,1.));
#29926=DIRECTION('ref_axis',(1.,0.,0.));
#29927=DIRECTION('',(0.,-1.,0.));
#29928=DIRECTION('',(1.,0.,0.));
#29929=DIRECTION('',(0.,1.,0.));
#29930=DIRECTION('',(-1.,0.,0.));
#29931=DIRECTION('',(-1.,0.,0.));
#29932=DIRECTION('',(-1.,0.,0.));
#29933=DIRECTION('center_axis',(0.,0.,1.));
#29934=DIRECTION('ref_axis',(1.,0.,0.));
#29935=DIRECTION('center_axis',(0.,0.,1.));
#29936=DIRECTION('ref_axis',(1.,0.,0.));
#29937=DIRECTION('',(0.,0.,1.));
#29938=DIRECTION('center_axis',(0.,0.,1.));
#29939=DIRECTION('ref_axis',(1.,0.,0.));
#29940=DIRECTION('center_axis',(0.,0.,1.));
#29941=DIRECTION('ref_axis',(1.,0.,0.));
#29942=DIRECTION('',(0.,0.,1.));
#29943=DIRECTION('center_axis',(0.,0.,1.));
#29944=DIRECTION('ref_axis',(1.,0.,0.));
#29945=DIRECTION('center_axis',(0.,0.,1.));
#29946=DIRECTION('ref_axis',(1.,0.,0.));
#29947=DIRECTION('',(0.,0.,1.));
#29948=DIRECTION('center_axis',(0.,0.,1.));
#29949=DIRECTION('ref_axis',(1.,0.,0.));
#29950=DIRECTION('center_axis',(0.,0.,1.));
#29951=DIRECTION('ref_axis',(1.,0.,0.));
#29952=DIRECTION('',(0.,0.,1.));
#29953=DIRECTION('center_axis',(0.,1.,0.));
#29954=DIRECTION('ref_axis',(-1.,0.,0.));
#29955=DIRECTION('',(-1.,0.,0.));
#29956=DIRECTION('',(0.,0.,1.));
#29957=DIRECTION('',(0.,0.,1.));
#29958=DIRECTION('center_axis',(1.,0.,0.));
#29959=DIRECTION('ref_axis',(0.,1.,0.));
#29960=DIRECTION('',(0.,1.,0.));
#29961=DIRECTION('',(0.,0.,1.));
#29962=DIRECTION('center_axis',(0.,-1.,0.));
#29963=DIRECTION('ref_axis',(1.,0.,0.));
#29964=DIRECTION('',(1.,0.,0.));
#29965=DIRECTION('',(0.,0.,1.));
#29966=DIRECTION('center_axis',(-1.,0.,0.));
#29967=DIRECTION('ref_axis',(0.,-1.,0.));
#29968=DIRECTION('',(0.,-1.,0.));
#29969=DIRECTION('center_axis',(0.,0.,1.));
#29970=DIRECTION('ref_axis',(1.,0.,0.));
#47976=CARTESIAN_POINT('',(0.,0.,0.));
#47977=CARTESIAN_POINT('Origin',(26.,-5.5,2.2));
#47978=CARTESIAN_POINT('',(25.5,-5.5,2.2));
#47979=CARTESIAN_POINT('',(25.5,-5.5,2.8));
#47980=CARTESIAN_POINT('',(25.5,-5.5,2.2));
#47981=CARTESIAN_POINT('',(26.,-5.,2.2));
#47982=CARTESIAN_POINT('Origin',(26.,-5.5,2.2));
#47983=CARTESIAN_POINT('',(26.,-5.,2.8));
#47984=CARTESIAN_POINT('',(26.,-5.,2.2));
#47985=CARTESIAN_POINT('Origin',(26.,-5.5,2.8));
#47986=CARTESIAN_POINT('Origin',(1.,-5.5,2.2));
#47987=CARTESIAN_POINT('',(0.5,-5.5,2.2));
#47988=CARTESIAN_POINT('',(0.5,-5.5,2.8));
#47989=CARTESIAN_POINT('',(0.5,-5.5,2.2));
#47990=CARTESIAN_POINT('',(1.,-5.,2.2));
#47991=CARTESIAN_POINT('Origin',(1.,-5.5,2.2));
#47992=CARTESIAN_POINT('',(1.,-5.,2.8));
#47993=CARTESIAN_POINT('',(1.,-5.,2.2));
#47994=CARTESIAN_POINT('Origin',(1.,-5.5,2.8));
#47995=CARTESIAN_POINT('Origin',(16.5,-6.,1.1));
#47996=CARTESIAN_POINT('',(16.335,-6.,1.2));
#47997=CARTESIAN_POINT('Origin',(16.5,-6.,1.2));
#47998=CARTESIAN_POINT('',(16.335,-6.,2.8));
#47999=CARTESIAN_POINT('',(16.335,-6.,1.1));
#48000=CARTESIAN_POINT('Origin',(16.5,-6.,2.8));
#48001=CARTESIAN_POINT('Origin',(10.5,-6.,1.1));
#48002=CARTESIAN_POINT('',(10.335,-6.,1.2));
#48003=CARTESIAN_POINT('Origin',(10.5,-6.,1.2));
#48004=CARTESIAN_POINT('',(10.335,-6.,2.8));
#48005=CARTESIAN_POINT('',(10.335,-6.,1.1));
#48006=CARTESIAN_POINT('Origin',(10.5,-6.,2.8));
#48007=CARTESIAN_POINT('Origin',(4.5,-6.,1.1));
#48008=CARTESIAN_POINT('',(4.335,-6.,1.2));
#48009=CARTESIAN_POINT('Origin',(4.5,-6.,1.2));
#48010=CARTESIAN_POINT('',(4.335,-6.,2.8));
#48011=CARTESIAN_POINT('',(4.335,-6.,1.1));
#48012=CARTESIAN_POINT('Origin',(4.5,-6.,2.8));
#48013=CARTESIAN_POINT('Origin',(22.5,-6.,1.1));
#48014=CARTESIAN_POINT('',(22.335,-6.,1.2));
#48015=CARTESIAN_POINT('Origin',(22.5,-6.,1.2));
#48016=CARTESIAN_POINT('',(22.335,-6.,2.8));
#48017=CARTESIAN_POINT('',(22.335,-6.,1.1));
#48018=CARTESIAN_POINT('Origin',(22.5,-6.,2.8));
#48019=CARTESIAN_POINT('Origin',(26.,-7.8,2.2));
#48020=CARTESIAN_POINT('',(25.5,-7.8,2.2));
#48021=CARTESIAN_POINT('Origin',(26.,-7.8,2.2));
#48022=CARTESIAN_POINT('',(25.5,-7.8,2.8));
#48023=CARTESIAN_POINT('',(25.5,-7.8,2.2));
#48024=CARTESIAN_POINT('Origin',(26.,-7.8,2.8));
#48025=CARTESIAN_POINT('Origin',(26.,-7.8,2.2));
#48026=CARTESIAN_POINT('',(25.725,-7.8,2.2));
#48027=CARTESIAN_POINT('Origin',(26.,-7.8,2.2));
#48028=CARTESIAN_POINT('Origin',(1.,-5.5,2.2));
#48029=CARTESIAN_POINT('Origin',(1.,-5.5,2.8));
#48030=CARTESIAN_POINT('',(1.,-5.,2.2));
#48031=CARTESIAN_POINT('Origin',(1.,-5.5,2.2));
#48032=CARTESIAN_POINT('Origin',(1.,-5.5,2.2));
#48033=CARTESIAN_POINT('',(0.725,-5.5,2.2));
#48034=CARTESIAN_POINT('Origin',(1.,-5.5,2.2));
#48035=CARTESIAN_POINT('Origin',(1.,-7.8,2.2));
#48036=CARTESIAN_POINT('',(0.5,-7.8,2.2));
#48037=CARTESIAN_POINT('Origin',(1.,-7.8,2.2));
#48038=CARTESIAN_POINT('',(0.5,-7.8,2.8));
#48039=CARTESIAN_POINT('',(0.5,-7.8,2.2));
#48040=CARTESIAN_POINT('Origin',(1.,-7.8,2.8));
#48041=CARTESIAN_POINT('Origin',(1.,-7.8,2.2));
#48042=CARTESIAN_POINT('',(0.725,-7.8,2.2));
#48043=CARTESIAN_POINT('Origin',(1.,-7.8,2.2));
#48044=CARTESIAN_POINT('Origin',(26.,-5.5,2.2));
#48045=CARTESIAN_POINT('Origin',(26.,-5.5,2.8));
#48046=CARTESIAN_POINT('',(26.,-5.,2.2));
#48047=CARTESIAN_POINT('Origin',(26.,-5.5,2.2));
#48048=CARTESIAN_POINT('Origin',(26.,-5.5,2.2));
#48049=CARTESIAN_POINT('',(25.725,-5.5,2.2));
#48050=CARTESIAN_POINT('Origin',(26.,-5.5,2.2));
#48051=CARTESIAN_POINT('Origin',(13.5,-6.75,2.8));
#48052=CARTESIAN_POINT('',(0.,-5.,2.8));
#48053=CARTESIAN_POINT('',(0.,-8.5,2.8));
#48054=CARTESIAN_POINT('',(0.,-5.,2.8));
#48055=CARTESIAN_POINT('',(27.,-8.5,2.8));
#48056=CARTESIAN_POINT('',(0.,-8.5,2.8));
#48057=CARTESIAN_POINT('',(27.,-5.,2.8));
#48058=CARTESIAN_POINT('',(27.,-8.5,2.8));
#48059=CARTESIAN_POINT('',(27.,-5.,2.8));
#48060=CARTESIAN_POINT('',(27.,-5.,2.8));
#48061=CARTESIAN_POINT('',(27.,-5.,2.8));
#48062=CARTESIAN_POINT('Origin',(26.,-7.8,1.1));
#48063=CARTESIAN_POINT('',(25.725,-7.8,1.2));
#48064=CARTESIAN_POINT('Origin',(26.,-7.8,1.2));
#48065=CARTESIAN_POINT('',(25.725,-7.8,1.1));
#48066=CARTESIAN_POINT('Origin',(1.,-5.5,1.1));
#48067=CARTESIAN_POINT('',(0.725,-5.5,1.2));
#48068=CARTESIAN_POINT('Origin',(1.,-5.5,1.2));
#48069=CARTESIAN_POINT('',(0.725,-5.5,1.1));
#48070=CARTESIAN_POINT('Origin',(1.,-7.8,1.1));
#48071=CARTESIAN_POINT('',(0.725,-7.8,1.2));
#48072=CARTESIAN_POINT('Origin',(1.,-7.8,1.2));
#48073=CARTESIAN_POINT('',(0.725,-7.8,1.1));
#48074=CARTESIAN_POINT('Origin',(26.,-5.5,1.1));
#48075=CARTESIAN_POINT('',(25.725,-5.5,1.2));
#48076=CARTESIAN_POINT('Origin',(26.,-5.5,1.2));
#48077=CARTESIAN_POINT('',(25.725,-5.5,1.1));
#48078=CARTESIAN_POINT('Origin',(27.,-5.,1.2));
#48079=CARTESIAN_POINT('',(27.,-5.,1.2));
#48080=CARTESIAN_POINT('',(0.,-5.,1.2));
#48081=CARTESIAN_POINT('',(27.,-5.,1.2));
#48082=CARTESIAN_POINT('',(0.,-5.,1.2));
#48083=CARTESIAN_POINT('',(27.,-5.,1.2));
#48084=CARTESIAN_POINT('Origin',(27.,-8.5,1.2));
#48085=CARTESIAN_POINT('',(27.,-8.5,1.2));
#48086=CARTESIAN_POINT('',(27.,-8.5,1.2));
#48087=CARTESIAN_POINT('',(27.,-8.5,1.2));
#48088=CARTESIAN_POINT('Origin',(0.,-8.5,1.2));
#48089=CARTESIAN_POINT('',(0.,-8.5,1.2));
#48090=CARTESIAN_POINT('',(0.,-8.5,1.2));
#48091=CARTESIAN_POINT('',(0.,-8.5,1.2));
#48092=CARTESIAN_POINT('Origin',(0.,-5.,1.2));
#48093=CARTESIAN_POINT('',(0.,-5.,1.2));
#48094=CARTESIAN_POINT('Origin',(13.5,-6.75,1.2));
#62840=UNCERTAINTY_MEASURE_WITH_UNIT(LENGTH_MEASURE(0.001),#62985,
'DISTANCE_ACCURACY_VALUE',
'Maximum model space distance between geometric entities at asserted c
onnectivities');
#62885=UNCERTAINTY_MEASURE_WITH_UNIT(LENGTH_MEASURE(0.001),#62985,
'DISTANCE_ACCURACY_VALUE',
'Maximum model space distance between geometric entities at asserted c
onnectivities');
#62939=(
GEOMETRIC_REPRESENTATION_CONTEXT(3)
GLOBAL_UNCERTAINTY_ASSIGNED_CONTEXT((#62840))
GLOBAL_UNIT_ASSIGNED_CONTEXT((#62985,#62987,#62988))
REPRESENTATION_CONTEXT('','3D')
);
#62984=(
GEOMETRIC_REPRESENTATION_CONTEXT(3)
GLOBAL_UNCERTAINTY_ASSIGNED_CONTEXT((#62885))
GLOBAL_UNIT_ASSIGNED_CONTEXT((#62985,#62987,#62988))
REPRESENTATION_CONTEXT('','3D')
);
#62985=(
LENGTH_UNIT()
NAMED_UNIT(*)
SI_UNIT(.CENTI.,.METRE.)
);
#62987=(
NAMED_UNIT(*)
PLANE_ANGLE_UNIT()
SI_UNIT($,.RADIAN.)
);
#62988=(
NAMED_UNIT(*)
SI_UNIT($,.STERADIAN.)
SOLID_ANGLE_UNIT()
);
#63042=SHAPE_DEFINITION_REPRESENTATION(#63220,#63402);
#63220=PRODUCT_DEFINITION_SHAPE('',$,#63501);
#63402=SHAPE_REPRESENTATION('',(#25299),#62939);
#63447=PRODUCT_DEFINITION_CONTEXT('part definition',#63743,'design');
#63501=PRODUCT_DEFINITION('Y Stage - 04 Rail adapter',
'Y Stage - 04 Rail adapter',#63599,#63447);
#63599=PRODUCT_DEFINITION_FORMATION('',$,#63798);
#63743=APPLICATION_CONTEXT(
'Core Data for Automotive Mechanical Design Process');
#63744=PRODUCT_CONTEXT('part definition',#63743,'mechanical');
#63798=PRODUCT('Y Stage - 04 Rail adapter','Y Stage - 04 Rail adapter',
'Y Stage - 04 Rail adapter',(#63744));
#63899=COLOUR_RGB('Sky Blue',0.24,0.69,0.87);
#63900=FILL_AREA_STYLE_COLOUR('',#63899);
#63901=FILL_AREA_STYLE('',(#63900));
#63902=SURFACE_STYLE_FILL_AREA(#63901);
#63903=SURFACE_SIDE_STYLE('',(#63902));
#63904=SURFACE_STYLE_USAGE(.BOTH.,#63903);
#63905=PRESENTATION_STYLE_ASSIGNMENT((#63904));
ENDSEC;
END-ISO-10303-21;
